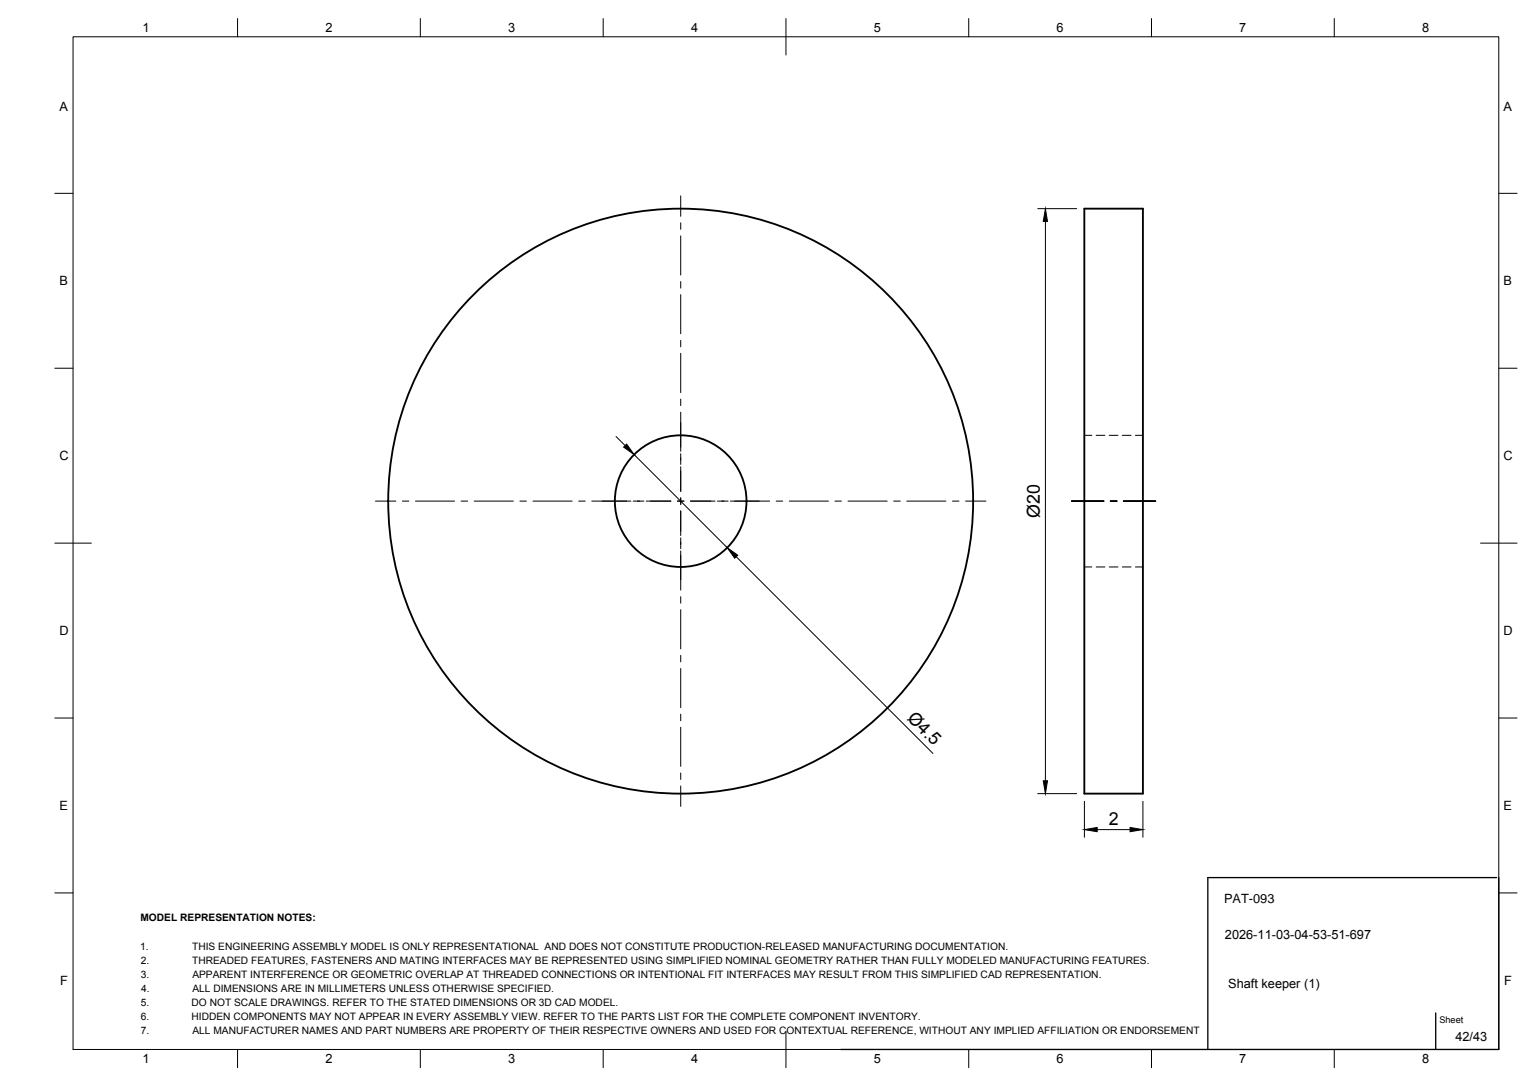
ISO-10303-21;
HEADER;
/* Generated by software containing ST-Developer
 * from STEP Tools, Inc. (www.steptools.com) 
 */

FILE_DESCRIPTION(
/* description */ ('Self-centering screw clamp'),
/* implementation_level */ '2;1');

FILE_NAME(
/* name */ 'Shaft keeper (1).step',
/* time_stamp */ '2026-10-28T03:25:31-07:00',
/* author */ (''),
/* organization */ (''),
/* preprocessor_version */ 'ST-DEVELOPER v20.2',
/* originating_system */ 'Autodesk Translation Framework v15.17.0.0',
/* authorisation */ '');

FILE_SCHEMA (('AUTOMOTIVE_DESIGN { 1 0 10303 214 3 1 1 }'));
ENDSEC;

DATA;
#10=MECHANICAL_DESIGN_GEOMETRIC_PRESENTATION_REPRESENTATION('',(#668),#16799);
#579=SHAPE_REPRESENTATION_RELATIONSHIP('SRR','None',#17057,#620);
#620=ADVANCED_BREP_SHAPE_REPRESENTATION('',(#715),#16795);
#668=STYLED_ITEM('',(#17326),#715);
#715=MANIFOLD_SOLID_BREP('Body1',#9120);
#1008=FACE_BOUND('',#2534,.T.);
#1009=FACE_BOUND('',#2536,.T.);
#1247=PLANE('',#10587);
#1248=PLANE('',#10588);
#1737=FACE_OUTER_BOUND('',#2531,.T.);
#1738=FACE_OUTER_BOUND('',#2532,.T.);
#1739=FACE_OUTER_BOUND('',#2533,.T.);
#1740=FACE_OUTER_BOUND('',#2535,.T.);
#2531=EDGE_LOOP('',(#8191,#8192,#8193,#8194));
#2532=EDGE_LOOP('',(#8195,#8196,#8197,#8198));
#2533=EDGE_LOOP('',(#8199));
#2534=EDGE_LOOP('',(#8200));
#2535=EDGE_LOOP('',(#8201));
#2536=EDGE_LOOP('',(#8202));
#3096=LINE('',#16358,#3669);
#3097=LINE('',#16364,#3670);
#3669=VECTOR('',#13283,0.225);
#3670=VECTOR('',#13290,1.);
#4211=CIRCLE('',#10582,0.225);
#4212=CIRCLE('',#10583,0.225);
#4213=CIRCLE('',#10585,1.);
#4214=CIRCLE('',#10586,1.);
#4923=VERTEX_POINT('',#16355);
#4924=VERTEX_POINT('',#16357);
#4925=VERTEX_POINT('',#16361);
#4926=VERTEX_POINT('',#16363);
#6020=EDGE_CURVE('',#4923,#4923,#4211,.T.);
#6021=EDGE_CURVE('',#4923,#4924,#3096,.T.);
#6022=EDGE_CURVE('',#4924,#4924,#4212,.T.);
#6023=EDGE_CURVE('',#4925,#4925,#4213,.T.);
#6024=EDGE_CURVE('',#4925,#4926,#3097,.T.);
#6025=EDGE_CURVE('',#4926,#4926,#4214,.T.);
#8191=ORIENTED_EDGE('',*,*,#6020,.F.);
#8192=ORIENTED_EDGE('',*,*,#6021,.T.);
#8193=ORIENTED_EDGE('',*,*,#6022,.T.);
#8194=ORIENTED_EDGE('',*,*,#6021,.F.);
#8195=ORIENTED_EDGE('',*,*,#6023,.F.);
#8196=ORIENTED_EDGE('',*,*,#6024,.T.);
#8197=ORIENTED_EDGE('',*,*,#6025,.T.);
#8198=ORIENTED_EDGE('',*,*,#6024,.F.);
#8199=ORIENTED_EDGE('',*,*,#6023,.T.);
#8200=ORIENTED_EDGE('',*,*,#6020,.T.);
#8201=ORIENTED_EDGE('',*,*,#6025,.F.);
#8202=ORIENTED_EDGE('',*,*,#6022,.F.);
#8563=CYLINDRICAL_SURFACE('',#10581,0.225);
#8564=CYLINDRICAL_SURFACE('',#10584,1.);
#9035=ADVANCED_FACE('',(#1737),#8563,.F.);
#9036=ADVANCED_FACE('',(#1738),#8564,.T.);
#9037=ADVANCED_FACE('',(#1739,#1008),#1247,.T.);
#9038=ADVANCED_FACE('',(#1740,#1009),#1248,.F.);
#9120=CLOSED_SHELL('',(#9035,#9036,#9037,#9038));
#10580=AXIS2_PLACEMENT_3D('',#16353,#13277,#13278);
#10581=AXIS2_PLACEMENT_3D('',#16354,#13279,#13280);
#10582=AXIS2_PLACEMENT_3D('',#16356,#13281,#13282);
#10583=AXIS2_PLACEMENT_3D('',#16359,#13284,#13285);
#10584=AXIS2_PLACEMENT_3D('',#16360,#13286,#13287);
#10585=AXIS2_PLACEMENT_3D('',#16362,#13288,#13289);
#10586=AXIS2_PLACEMENT_3D('',#16365,#13291,#13292);
#10587=AXIS2_PLACEMENT_3D('',#16366,#13293,#13294);
#10588=AXIS2_PLACEMENT_3D('',#16367,#13295,#13296);
#13277=DIRECTION('axis',(0.,0.,1.));
#13278=DIRECTION('refdir',(1.,0.,0.));
#13279=DIRECTION('center_axis',(1.,0.,0.));
#13280=DIRECTION('ref_axis',(0.,0.,-1.));
#13281=DIRECTION('center_axis',(-1.,0.,0.));
#13282=DIRECTION('ref_axis',(0.,0.,-1.));
#13283=DIRECTION('',(-1.,0.,0.));
#13284=DIRECTION('center_axis',(-1.,0.,0.));
#13285=DIRECTION('ref_axis',(0.,0.,-1.));
#13286=DIRECTION('center_axis',(1.,0.,0.));
#13287=DIRECTION('ref_axis',(0.,0.,-1.));
#13288=DIRECTION('center_axis',(1.,0.,0.));
#13289=DIRECTION('ref_axis',(0.,0.,-1.));
#13290=DIRECTION('',(-1.,0.,0.));
#13291=DIRECTION('center_axis',(1.,0.,0.));
#13292=DIRECTION('ref_axis',(0.,0.,-1.));
#13293=DIRECTION('center_axis',(1.,0.,0.));
#13294=DIRECTION('ref_axis',(0.,0.,-1.));
#13295=DIRECTION('center_axis',(1.,0.,0.));
#13296=DIRECTION('ref_axis',(0.,0.,-1.));
#16353=CARTESIAN_POINT('',(0.,0.,0.));
#16354=CARTESIAN_POINT('Origin',(14.5,0.,4.));
#16355=CARTESIAN_POINT('',(14.7,-2.75545529808155E-17,4.225));
#16356=CARTESIAN_POINT('Origin',(14.7,0.,4.));
#16357=CARTESIAN_POINT('',(14.5,-2.75545529808155E-17,4.225));
#16358=CARTESIAN_POINT('',(14.5,-2.75545529808155E-17,4.225));
#16359=CARTESIAN_POINT('Origin',(14.5,0.,4.));
#16360=CARTESIAN_POINT('Origin',(14.5,0.,4.));
#16361=CARTESIAN_POINT('',(14.7,-1.22464679914735E-16,5.));
#16362=CARTESIAN_POINT('Origin',(14.7,0.,4.));
#16363=CARTESIAN_POINT('',(14.5,-1.22464679914735E-16,5.));
#16364=CARTESIAN_POINT('',(14.5,-1.22464679914735E-16,5.));
#16365=CARTESIAN_POINT('Origin',(14.5,0.,4.));
#16366=CARTESIAN_POINT('Origin',(14.7,0.,4.));
#16367=CARTESIAN_POINT('Origin',(14.5,0.,4.));
#16746=UNCERTAINTY_MEASURE_WITH_UNIT(LENGTH_MEASURE(0.001),#16800,
'DISTANCE_ACCURACY_VALUE',
'Maximum model space distance between geometric entities at asserted c
onnectivities');
#16750=UNCERTAINTY_MEASURE_WITH_UNIT(LENGTH_MEASURE(0.001),#16800,
'DISTANCE_ACCURACY_VALUE',
'Maximum model space distance between geometric entities at asserted c
onnectivities');
#16795=(
GEOMETRIC_REPRESENTATION_CONTEXT(3)
GLOBAL_UNCERTAINTY_ASSIGNED_CONTEXT((#16746))
GLOBAL_UNIT_ASSIGNED_CONTEXT((#16800,#16802,#16803))
REPRESENTATION_CONTEXT('','3D')
);
#16799=(
GEOMETRIC_REPRESENTATION_CONTEXT(3)
GLOBAL_UNCERTAINTY_ASSIGNED_CONTEXT((#16750))
GLOBAL_UNIT_ASSIGNED_CONTEXT((#16800,#16802,#16803))
REPRESENTATION_CONTEXT('','3D')
);
#16800=(
LENGTH_UNIT()
NAMED_UNIT(*)
SI_UNIT(.CENTI.,.METRE.)
);
#16802=(
NAMED_UNIT(*)
PLANE_ANGLE_UNIT()
SI_UNIT($,.RADIAN.)
);
#16803=(
NAMED_UNIT(*)
SI_UNIT($,.STERADIAN.)
SOLID_ANGLE_UNIT()
);
#16848=SHAPE_DEFINITION_REPRESENTATION(#16903,#17057);
#16903=PRODUCT_DEFINITION_SHAPE('',$,#17106);
#17057=SHAPE_REPRESENTATION('',(#10580),#16795);
#17061=PRODUCT_DEFINITION_CONTEXT('part definition',#17207,'design');
#17106=PRODUCT_DEFINITION('Shaft keeper (1)','Shaft keeper (1)',#17154,#17061);
#17154=PRODUCT_DEFINITION_FORMATION('',$,#17253);
#17207=APPLICATION_CONTEXT(
'Core Data for Automotive Mechanical Design Process');
#17208=PRODUCT_CONTEXT('part definition',#17207,'mechanical');
#17253=PRODUCT('Shaft keeper (1)','Shaft keeper (1)','Shaft keeper (1)',(#17208));
#17320=COLOUR_RGB('Grey',0.48,0.52,0.57);
#17321=FILL_AREA_STYLE_COLOUR('',#17320);
#17322=FILL_AREA_STYLE('',(#17321));
#17323=SURFACE_STYLE_FILL_AREA(#17322);
#17324=SURFACE_SIDE_STYLE('',(#17323));
#17325=SURFACE_STYLE_USAGE(.BOTH.,#17324);
#17326=PRESENTATION_STYLE_ASSIGNMENT((#17325));
ENDSEC;
END-ISO-10303-21;
